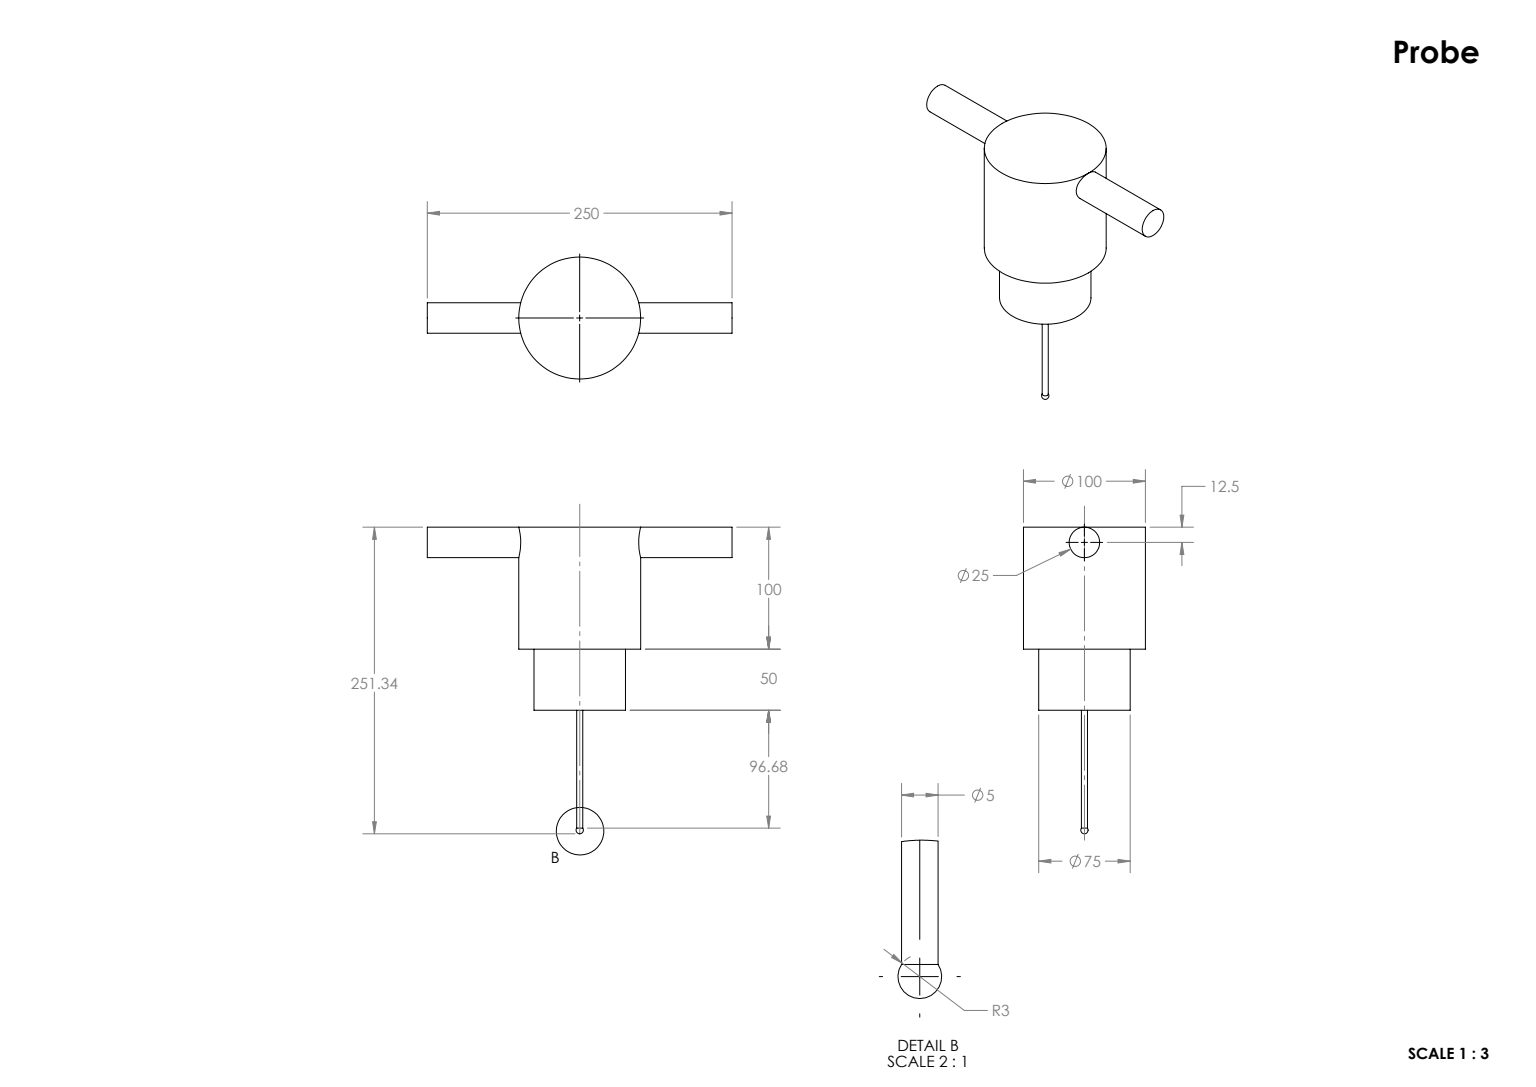
ISO-10303-21;
HEADER;
FILE_DESCRIPTION (('STEP AP214'),
    '1' );
FILE_NAME ('Probe.step',
    '2026-10-28T15:55:38',
    ( '' ),
    ( '' ),
    'SwSTEP 2.0',
    'SolidWorks 2025',
    '' );
FILE_SCHEMA (( 'AUTOMOTIVE_DESIGN' ));
ENDSEC;

DATA;
#19=ADVANCED_FACE ( 'NONE', ( #8129 ), #7501, .T. ) ;
#39=CARTESIAN_POINT ( 'NONE',  ( 0.000000000000000000, 7.945337353457666419E-16, -150.0000000000000000 ) ) ;
#48=VERTEX_POINT ( 'NONE', #4805 ) ;
#114=CARTESIAN_POINT ( 'NONE',  ( -0.8292248493948853882, 50.00000000000000000, -1.010867942207665278E-14 ) ) ;
#115=FACE_OUTER_BOUND ( 'NONE', #7634, .T. ) ;
#118=DIRECTION ( 'NONE',  ( 0.000000000000000000, 0.000000000000000000, -1.000000000000000000 ) ) ;
#135=EDGE_CURVE ( 'NONE', #3598, #1656, #3145, .T. ) ;
#154=CARTESIAN_POINT ( 'NONE',  ( -5.558076868459232323, 49.69586384218322905, -1.274058936613796877 ) ) ;
#176=LINE ( 'NONE', #2239, #1981 ) ;
#182=ORIENTED_EDGE ( 'NONE', *, *, #917, .F. ) ;
#188=ADVANCED_FACE ( 'NONE', ( #4425 ), #4987, .T. ) ;
#201=DIRECTION ( 'NONE',  ( 0.000000000000000000, -0.000000000000000000, 1.000000000000000000 ) ) ;
#222=AXIS2_PLACEMENT_3D ( 'NONE', #4618, #3222, #5811 ) ;
#242=CARTESIAN_POINT ( 'NONE',  ( 8.253058034503027329, 49.31520865873546455, -3.102932425833026642 ) ) ;
#263=DIRECTION ( 'NONE',  ( -0.000000000000000000, -7.945337353457666666E-18, -1.000000000000000000 ) ) ;
#281=CARTESIAN_POINT ( 'NONE',  ( 0.000000000000000000, 50.00000000000000000, 0.000000000000000000 ) ) ;
#307=PLANE ( 'NONE',  #7987 ) ;
#327=CARTESIAN_POINT ( 'NONE',  ( 11.38744771879169093, 48.68625849413228934, -7.328777110660809946 ) ) ;
#334=VERTEX_POINT ( 'NONE', #4039 ) ;
#341=CARTESIAN_POINT ( 'NONE',  ( -8.253058034503022000, -49.31520865873545034, -3.102932425833025309 ) ) ;
#392=ORIENTED_EDGE ( 'NONE', *, *, #1590, .F. ) ;
#401=CARTESIAN_POINT ( 'NONE',  ( 1.632468168883557169, -49.97996006834705440, -24.92059050027006606 ) ) ;
#418=ORIENTED_EDGE ( 'NONE', *, *, #1413, .T. ) ;
#423=CARTESIAN_POINT ( 'NONE',  ( 0.000000000000000000, 1.191800603018649864E-15, -100.0000000000000000 ) ) ;
#435=EDGE_LOOP ( 'NONE', ( #3516, #6927 ) ) ;
#446=ORIENTED_EDGE ( 'NONE', *, *, #1545, .T. ) ;
#457=AXIS2_PLACEMENT_3D ( 'NONE', #8109, #6795, #201 ) ;
#479=CARTESIAN_POINT ( 'NONE',  ( -11.83759003446072811, -48.57866412327431505, -8.463974912767858072 ) ) ;
#484=CARTESIAN_POINT ( 'NONE',  ( 0.000000000000000000, 37.49999999999999289, -150.0000000000000000 ) ) ;
#491=UNCERTAINTY_MEASURE_WITH_UNIT (LENGTH_MEASURE( 1.000000000000000082E-05 ), #6982, 'distance_accuracy_value', 'NONE');
#496=ADVANCED_FACE ( 'NONE', ( #6675 ), #5448, .T. ) ;
#505=EDGE_CURVE ( 'NONE', #48, #4486, #8022, .T. ) ;
#522=CARTESIAN_POINT ( 'NONE',  ( -3.257728639534228865, -49.90026920665918198, -24.59591892738197672 ) ) ;
#526=CARTESIAN_POINT ( 'NONE',  ( 0.000000000000000000, 7.945337353457666419E-16, -150.0000000000000000 ) ) ;
#533=CARTESIAN_POINT ( 'NONE',  ( 11.22541203495697104, -48.72469304432832615, -18.06039341770851436 ) ) ;
#551=CARTESIAN_POINT ( 'NONE',  ( 12.41819479434714069, 48.43362276422629975, -14.14586790793774895 ) ) ;
#558=CARTESIAN_POINT ( 'NONE',  ( -9.403142016537936243, 49.10855715295182478, -4.253968596005561764 ) ) ;
#573=SHAPE_REPRESENTATION ( 'Probe', ( #1299 ), #7094 ) ;
#575=CARTESIAN_POINT ( 'NONE',  ( 9.403142016537936243, -49.10855715295183188, -4.253968596005562652 ) ) ;
#592=CARTESIAN_POINT ( 'NONE',  ( 4.037232620646171277, 49.84250566375262537, -24.35825330067164884 ) ) ;
#595=DIRECTION ( 'NONE',  ( 0.000000000000000000, 1.000000000000000000, 0.000000000000000000 ) ) ;
#618=CARTESIAN_POINT ( 'NONE',  ( 12.39753912377990552, -48.43864980223353456, -14.14916085730400219 ) ) ;
#640=DIRECTION ( 'NONE',  ( 0.000000000000000000, -7.945337353457666666E-18, -1.000000000000000000 ) ) ;
#658=CARTESIAN_POINT ( 'NONE',  ( 10.16267929626374489, -48.95685099404312979, -19.78936650929338725 ) ) ;
#661=FACE_OUTER_BOUND ( 'NONE', #6204, .T. ) ;
#662=ORIENTED_EDGE ( 'NONE', *, *, #737, .F. ) ;
#680=EDGE_CURVE ( 'NONE', #1656, #1706, #2751, .T. ) ;
#702=CARTESIAN_POINT ( 'NONE',  ( 6.614448519079572542, -49.56174273647120998, -23.11440585317444985 ) ) ;
#721=EDGE_CURVE ( 'NONE', #7126, #7967, #3963, .T. ) ;
#737=EDGE_CURVE ( 'NONE', #986, #5147, #4224, .T. ) ;
#739=ORIENTED_EDGE ( 'NONE', *, *, #1590, .T. ) ;
#742=VECTOR ( 'NONE', #864, 1000.000000000000000 ) ;
#775=ORIENTED_EDGE ( 'NONE', *, *, #5713, .F. ) ;
#781=DIRECTION ( 'NONE',  ( -0.000000000000000000, -7.945337353457666666E-18, -1.000000000000000000 ) ) ;
#791=DIRECTION ( 'NONE',  ( 0.000000000000000000, 1.000000000000000000, -7.945337353457666666E-18 ) ) ;
#843=EDGE_LOOP ( 'NONE', ( #1832, #4978 ) ) ;
#856=ORIENTED_EDGE ( 'NONE', *, *, #2130, .F. ) ;
#861=DIRECTION ( 'NONE',  ( 0.000000000000000000, 0.000000000000000000, -1.000000000000000000 ) ) ;
#864=DIRECTION ( 'NONE',  ( -0.000000000000000000, -7.945337353457666666E-18, -1.000000000000000000 ) ) ;
#908=CARTESIAN_POINT ( 'NONE',  ( 6.123233995736765296E-15, -49.99999999999999289, -250.0000000000000000 ) ) ;
#917=EDGE_CURVE ( 'NONE', #6329, #7967, #176, .T. ) ;
#918=AXIS2_PLACEMENT_3D ( 'NONE', #7982, #6026, #118 ) ;
#936=CARTESIAN_POINT ( 'NONE',  ( 9.415432556623352767, 49.10895683582204896, -4.238112224658974192 ) ) ;
#941=DIRECTION ( 'NONE',  ( -0.000000000000000000, -7.945337353457666666E-18, -1.000000000000000000 ) ) ;
#986=VERTEX_POINT ( 'NONE', #3576 ) ;
#987=AXIS2_PLACEMENT_3D ( 'NONE', #3005, #4347, #3590 ) ;
#993=CARTESIAN_POINT ( 'NONE',  ( -3.243174531372579494, -49.89626761698126245, -0.4210505255250470702 ) ) ;
#996=ORIENTED_EDGE ( 'NONE', *, *, #4675, .T. ) ;
#997=DIRECTION ( 'NONE',  ( -0.000000000000000000, -7.945337353457666666E-18, -1.000000000000000000 ) ) ;
#1024=EDGE_CURVE ( 'NONE', #3915, #6928, #8311, .T. ) ;
#1028=AXIS2_PLACEMENT_3D ( 'NONE', #3244, #2009, #3886 ) ;
#1035=DIRECTION ( 'NONE',  ( 0.000000000000000000, 1.000000000000000000, 0.000000000000000000 ) ) ;
#1043=CARTESIAN_POINT ( 'NONE',  ( 6.123246359811209136E-15, -49.99999999999999289, -25.00000000000000000 ) ) ;
#1058=CARTESIAN_POINT ( 'NONE',  ( 10.82846484896509409, 48.81376096915064267, -6.242155733168283760 ) ) ;
#1069=ORIENTED_EDGE ( 'NONE', *, *, #2887, .T. ) ;
#1072=CIRCLE ( 'NONE', #2296, 49.99999999999998579 ) ;
#1077=CARTESIAN_POINT ( 'NONE',  ( -6.271675211807169248, -49.60982880777383741, -1.656483108071704846 ) ) ;
#1130=DIRECTION ( 'NONE',  ( -0.000000000000000000, -7.945337353457666666E-18, -1.000000000000000000 ) ) ;
#1150=ORIENTED_EDGE ( 'NONE', *, *, #1915, .F. ) ;
#1154=CARTESIAN_POINT ( 'NONE',  ( -12.41973075191816633, 48.43322590808264039, -10.86594944112156291 ) ) ;
#1157=ADVANCED_FACE ( 'NONE', ( #2546 ), #4549, .F. ) ;
#1171=CARTESIAN_POINT ( 'NONE',  ( 8.557270319823464533, -49.26314968593496957, -3.379276828450694214 ) ) ;
#1190=CIRCLE ( 'NONE', #5890, 37.49999999999999289 ) ;
#1198=CARTESIAN_POINT ( 'NONE',  ( -12.10063575899649813, 48.51393303002350166, -9.260486547765557575 ) ) ;
#1203=FACE_OUTER_BOUND ( 'NONE', #1797, .T. ) ;
#1234=EDGE_LOOP ( 'NONE', ( #2994, #6172, #2615, #1150, #7419, #6336 ) ) ;
#1237=ADVANCED_FACE ( 'NONE', ( #115 ), #2704, .T. ) ;
#1240=CARTESIAN_POINT ( 'NONE',  ( -8.256742446866505603, 49.31458024324043521, -3.106261761854182790 ) ) ;
#1254=AXIS2_PLACEMENT_3D ( 'NONE', #7140, #640, #1365 ) ;
#1256=DIRECTION ( 'NONE',  ( -0.000000000000000000, -7.945337353457666666E-18, -1.000000000000000000 ) ) ;
#1274=CARTESIAN_POINT ( 'NONE',  ( -11.69966253144281332, 48.61218256317027198, -16.92010850872651417 ) ) ;
#1299=AXIS2_PLACEMENT_3D ( 'NONE', #5884, #1507, #5927 ) ;
#1319=DIRECTION ( 'NONE',  ( 0.000000000000000000, 1.000000000000000000, -7.945337353457666666E-18 ) ) ;
#1320=DIRECTION ( 'NONE',  ( -0.000000000000000000, -7.945337353457666666E-18, -1.000000000000000000 ) ) ;
#1330=CIRCLE ( 'NONE', #1730, 37.50000000000000000 ) ;
#1333=AXIS2_PLACEMENT_3D ( 'NONE', #3199, #3801, #595 ) ;
#1336=CARTESIAN_POINT ( 'NONE',  ( 3.061616997868370815E-16, -2.499999999999990230, -250.0000000000000000 ) ) ;
#1365=DIRECTION ( 'NONE',  ( 0.000000000000000000, 1.000000000000000000, -7.945337353457666666E-18 ) ) ;
#1384=DIRECTION ( 'NONE',  ( 0.000000000000000000, 1.000000000000000000, 0.000000000000000000 ) ) ;
#1412=VECTOR ( 'NONE', #1613, 1000.000000000000000 ) ;
#1413=EDGE_CURVE ( 'NONE', #5147, #4486, #4874, .T. ) ;
#1437=ADVANCED_FACE ( 'NONE', ( #7243, #6733 ), #307, .T. ) ;
#1502=FACE_OUTER_BOUND ( 'NONE', #1234, .T. ) ;
#1507=DIRECTION ( 'NONE',  ( 0.000000000000000000, 0.000000000000000000, 1.000000000000000000 ) ) ;
#1524=CARTESIAN_POINT ( 'NONE',  ( -6.274835263354055392, 49.60946935866542162, -1.658027691731842168 ) ) ;
#1527=DIRECTION ( 'NONE',  ( 0.000000000000000000, 1.000000000000000000, 0.000000000000000000 ) ) ;
#1540=DIRECTION ( 'NONE',  ( 0.000000000000000000, 1.000000000000000000, 0.000000000000000000 ) ) ;
#1545=EDGE_CURVE ( 'NONE', #6928, #3915, #4197, .T. ) ;
#1582=CARTESIAN_POINT ( 'NONE',  ( -11.21042436406065868, -48.72746226073034137, -18.04468079945885250 ) ) ;
#1590=EDGE_CURVE ( 'NONE', #4209, #6887, #3943, .T. ) ;
#1613=DIRECTION ( 'NONE',  ( -0.000000000000000000, -1.000000000000000000, -0.000000000000000000 ) ) ;
#1627=CARTESIAN_POINT ( 'NONE',  ( -0.8294483708339484007, -50.00000000000000711, -7.623296525288703052E-18 ) ) ;
#1641=ORIENTED_EDGE ( 'NONE', *, *, #4698, .F. ) ;
#1653=CARTESIAN_POINT ( 'NONE',  ( 0.000000000000000000, -125.0000000000000000, -12.50000000000000000 ) ) ;
#1655=EDGE_CURVE ( 'NONE', #6306, #986, #7595, .T. ) ;
#1656=VERTEX_POINT ( 'NONE', #5197 ) ;
#1706=VERTEX_POINT ( 'NONE', #4397 ) ;
#1707=CARTESIAN_POINT ( 'NONE',  ( -12.09737906851130518, -48.51474822866212122, -15.75174765218248574 ) ) ;
#1730=AXIS2_PLACEMENT_3D ( 'NONE', #423, #3269, #2425 ) ;
#1746=EDGE_LOOP ( 'NONE', ( #2201, #2378 ) ) ;
#1747=EDGE_LOOP ( 'NONE', ( #5047, #7771, #6216, #6700 ) ) ;
#1770=CARTESIAN_POINT ( 'NONE',  ( 6.260380647299085055, -49.60786550102538683, -23.32709356835264103 ) ) ;
#1772=CARTESIAN_POINT ( 'NONE',  ( 0.000000000000000000, 0.000000000000000000, -248.3416876048222832 ) ) ;
#1781=CARTESIAN_POINT ( 'NONE',  ( 9.126495132297687718, 49.16089547422080130, -21.05129937300930010 ) ) ;
#1797=EDGE_LOOP ( 'NONE', ( #6153, #2426, #2650, #2275 ) ) ;
#1798=CARTESIAN_POINT ( 'NONE',  ( -0.4088724290315628451, -49.99999999999999289, -25.00000000000000000 ) ) ;
#1813=SPHERICAL_SURFACE ( 'NONE', #3588, 3.000000000000001776 ) ;
#1832=ORIENTED_EDGE ( 'NONE', *, *, #6250, .F. ) ;
#1835=CARTESIAN_POINT ( 'NONE',  ( -9.920070434648176061, 49.00675803034337008, -20.11641848348689976 ) ) ;
#1838=DIRECTION ( 'NONE',  ( 0.000000000000000000, 0.000000000000000000, -1.000000000000000000 ) ) ;
#1846=CARTESIAN_POINT ( 'NONE',  ( 12.10063575899649990, -48.51393303002349455, -9.260486547765564680 ) ) ;
#1865=CARTESIAN_POINT ( 'NONE',  ( 7.630101673356683101, 49.41909675622682840, -22.43442449636368252 ) ) ;
#1879=CARTESIAN_POINT ( 'NONE',  ( -6.260380647299085055, 49.60786550102537973, -23.32709356835263748 ) ) ;
#1881=CIRCLE ( 'NONE', #1333, 2.499999999999984013 ) ;
#1885=DIRECTION ( 'NONE',  ( -0.000000000000000000, -1.000000000000000000, -0.000000000000000000 ) ) ;
#1888=CARTESIAN_POINT ( 'NONE',  ( 0.000000000000000000, -1.262567713204993255E-33, -150.0000000000000000 ) ) ;
#1890=CARTESIAN_POINT ( 'NONE',  ( -10.16275934324372265, -48.95683464664497819, -19.78926114801198821 ) ) ;
#1895=CYLINDRICAL_SURFACE ( 'NONE', #4148, 37.49999999999999289 ) ;
#1896=CARTESIAN_POINT ( 'NONE',  ( 12.07731880710695904, -48.51961889015784379, -15.74894529186713577 ) ) ;
#1912=CARTESIAN_POINT ( 'NONE',  ( 0.4088724290315675081, 49.99999999999999289, -24.99999999999999645 ) ) ;
#1915=EDGE_CURVE ( 'NONE', #6329, #6306, #3408, .T. ) ;
#1923=CARTESIAN_POINT ( 'NONE',  ( -9.123515037571456432, 49.16144051280856786, -21.05438506594878945 ) ) ;
#1947=CARTESIAN_POINT ( 'NONE',  ( 0.000000000000000000, -125.0000000000000000, -12.50000000000000000 ) ) ;
#1957=CARTESIAN_POINT ( 'NONE',  ( 12.50034226774477730, 48.41220345444930473, -13.31371842734950839 ) ) ;
#1971=LINE ( 'NONE', #3126, #6847 ) ;
#1975=CARTESIAN_POINT ( 'NONE',  ( -8.257771144136533792, -49.31688802671483529, -21.91964719072836232 ) ) ;
#1981=VECTOR ( 'NONE', #4658, 1000.000000000000000 ) ;
#2009=DIRECTION ( 'NONE',  ( 0.000000000000000000, 1.000000000000000000, 0.000000000000000000 ) ) ;
#2027=AXIS2_PLACEMENT_3D ( 'NONE', #3385, #5895, #2157 ) ;
#2037=AXIS2_PLACEMENT_3D ( 'NONE', #3347, #2118, #2154 ) ;
#2043=VECTOR ( 'NONE', #2971, 1000.000000000000000 ) ;
#2071=EDGE_LOOP ( 'NONE', ( #4525, #6589, #7855 ) ) ;
#2090=AXIS2_PLACEMENT_3D ( 'NONE', #4600, #2777, #1319 ) ;
#2118=DIRECTION ( 'NONE',  ( -0.000000000000000000, -7.945337353457666666E-18, -1.000000000000000000 ) ) ;
#2130=EDGE_CURVE ( 'NONE', #6306, #6329, #5453, .T. ) ;
#2143=CARTESIAN_POINT ( 'NONE',  ( 0.000000000000000000, 0.000000000000000000, -250.0000000000000000 ) ) ;
#2154=DIRECTION ( 'NONE',  ( 0.000000000000000000, 1.000000000000000000, -7.945337353457666666E-18 ) ) ;
#2157=DIRECTION ( 'NONE',  ( 0.000000000000000000, 0.000000000000000000, -1.000000000000000000 ) ) ;
#2185=DIRECTION ( 'NONE',  ( -0.000000000000000000, -1.000000000000000000, -0.000000000000000000 ) ) ;
#2201=ORIENTED_EDGE ( 'NONE', *, *, #135, .F. ) ;
#2213=DIRECTION ( 'NONE',  ( -0.000000000000000000, -7.945337353457666666E-18, -1.000000000000000000 ) ) ;
#2236=CARTESIAN_POINT ( 'NONE',  ( -12.41819479434713891, -48.43362276422628554, -14.14586790793774895 ) ) ;
#2237=SHAPE_REPRESENTATION_RELATIONSHIP ( 'NONE' , 'NONE' ,  #573, #6521 ) ;
#2239=CARTESIAN_POINT ( 'NONE',  ( 0.000000000000000000, 49.99999999999999289, -250.0000000000000000 ) ) ;
#2250=CARTESIAN_POINT ( 'NONE',  ( 0.000000000000000000, 1.191800603018649864E-15, -100.0000000000000000 ) ) ;
#2256=DIRECTION ( 'NONE',  ( 1.000000000000000000, -0.000000000000000000, 0.000000000000000000 ) ) ;
#2275=ORIENTED_EDGE ( 'NONE', *, *, #7081, .F. ) ;
#2296=AXIS2_PLACEMENT_3D ( 'NONE', #6352, #1256, #5080 ) ;
#2310=CARTESIAN_POINT ( 'NONE',  ( -12.07658505203027843, -48.51980254810341364, -9.248211290718611366 ) ) ;
#2350=CARTESIAN_POINT ( 'NONE',  ( -2.846087801003401196, -49.92054308009031161, -0.3214687869884009230 ) ) ;
#2351=( LENGTH_UNIT ( ) NAMED_UNIT ( * ) SI_UNIT ( .MILLI., .METRE. ) );
#2378=ORIENTED_EDGE ( 'NONE', *, *, #2977, .F. ) ;
#2391=CARTESIAN_POINT ( 'NONE',  ( -8.554558110533214688, -49.26362287191481215, -3.376715202643650215 ) ) ;
#2414=AXIS2_PLACEMENT_3D ( 'NONE', #3771, #1320, #7059 ) ;
#2418=CARTESIAN_POINT ( 'NONE',  ( 5.169052467613985513, 49.73353547763981908, -23.88849205255369412 ) ) ;
#2425=DIRECTION ( 'NONE',  ( 0.000000000000000000, 1.000000000000000000, 0.000000000000000000 ) ) ;
#2426=ORIENTED_EDGE ( 'NONE', *, *, #680, .T. ) ;
#2462=CARTESIAN_POINT ( 'NONE',  ( 12.07658505203027843, 48.51980254810342075, -9.248211290718606037 ) ) ;
#2470=DIRECTION ( 'NONE',  ( -0.000000000000000000, -7.945337353457666666E-18, -1.000000000000000000 ) ) ;
#2486=CARTESIAN_POINT ( 'NONE',  ( 9.123515037571451103, -49.16144051280858207, -21.05438506594878234 ) ) ;
#2501=CARTESIAN_POINT ( 'NONE',  ( 12.41960978562214102, 48.43326235599739960, -10.86247626165360813 ) ) ;
#2506=CARTESIAN_POINT ( 'NONE',  ( -11.83910760917652460, 48.57829327830486221, -16.53147691254502760 ) ) ;
#2507=ORIENTED_EDGE ( 'NONE', *, *, #5064, .T. ) ;
#2546=FACE_OUTER_BOUND ( 'NONE', #6856, .T. ) ;
#2563=CARTESIAN_POINT ( 'NONE',  ( 9.920070434648168956, -49.00675803034337719, -20.11641848348691042 ) ) ;
#2564=VECTOR ( 'NONE', #6472, 1000.000000000000000 ) ;
#2578=ADVANCED_FACE ( 'NONE', ( #4354 ), #1813, .T. ) ;
#2581=CARTESIAN_POINT ( 'NONE',  ( 10.16275934324372621, 48.95683464664498530, -19.78926114801199532 ) ) ;
#2598=CARTESIAN_POINT ( 'NONE',  ( -0.8183949479883554368, -49.99498560413270809, -24.97998898815200874 ) ) ;
#2615=ORIENTED_EDGE ( 'NONE', *, *, #5679, .T. ) ;
#2643=CARTESIAN_POINT ( 'NONE',  ( 8.258796090566862702, -49.31668406204209276, -21.91840799305901299 ) ) ;
#2647=ORIENTED_EDGE ( 'NONE', *, *, #8043, .T. ) ;
#2650=ORIENTED_EDGE ( 'NONE', *, *, #8282, .F. ) ;
#2690=DIRECTION ( 'NONE',  ( -1.000000000000000000, -1.224646799147353207E-16, 9.730231958057834423E-34 ) ) ;
#2692=CIRCLE ( 'NONE', #3349, 12.50000000000000000 ) ;
#2694=FACE_OUTER_BOUND ( 'NONE', #3875, .T. ) ;
#2698=VECTOR ( 'NONE', #7949, 1000.000000000000000 ) ;
#2704=CYLINDRICAL_SURFACE ( 'NONE', #6225, 2.499999999999990230 ) ;
#2710=ORIENTED_EDGE ( 'NONE', *, *, #6560, .T. ) ;
#2715=ADVANCED_FACE ( 'NONE', ( #661 ), #7879, .T. ) ;
#2751=LINE ( 'NONE', #7916, #742 ) ;
#2761=EDGE_LOOP ( 'NONE', ( #662, #5308, #3301, #6052 ) ) ;
#2777=DIRECTION ( 'NONE',  ( -0.000000000000000000, -7.945337353457666666E-18, -1.000000000000000000 ) ) ;
#2786=ORIENTED_EDGE ( 'NONE', *, *, #4582, .F. ) ;
#2803=VERTEX_POINT ( 'NONE', #7962 ) ;
#2820=CARTESIAN_POINT ( 'NONE',  ( 8.554558110533218240, 49.26362287191481926, -3.376715202643651992 ) ) ;
#2830=B_SPLINE_CURVE_WITH_KNOTS ( 'NONE', 3,
 ( #1043, #3597, #401, #7500, #4263, #6264, #3644, #1770, #702, #5767, #2643, #2486, #5683, #2563, #658, #4481, #533, #7033, #6353, #1896, #4352, #6426, #618, #5126, #7071, #3258, #3218, #1846, #5848, #5081, #7116, #3177, #5212, #575, #3784, #1171, #5809, #7726, #3736, #7631, #3106, #7764, #6313, #5043, #8266, #4440, #4391, #3860 ),
 .UNSPECIFIED., .F., .F.,
 ( 4, 2, 2, 2, 2, 2, 2, 2, 2, 2, 2, 2, 2, 2, 2, 2, 2, 2, 2, 2, 2, 2, 2, 4 ),
 ( 0.03923685324657889828, 0.04168849572278653104, 0.04414013819899415686, 0.04536595943709797324, 0.04659178067520178962, 0.04904342315140942932, 0.05026924438951324570, 0.05149506562761706902, 0.05394670810382472259, 0.05517252934192855285, 0.05639835058003237617, 0.05762417181813619949, 0.05884999305624002280, 0.06130163553244767638, 0.06375327800865532302, 0.06620492048486296965, 0.06743074172296678603, 0.06865656296107061629, 0.06988238419917444655, 0.07110820543727826293, 0.07355984791348590957, 0.07478566915158973982, 0.07601149038969357008, 0.07846313286590121672 ),
 .UNSPECIFIED. ) ;
#2875=LINE ( 'NONE', #908, #4393 ) ;
#2887=EDGE_CURVE ( 'NONE', #48, #7126, #2875, .T. ) ;
#2896=CARTESIAN_POINT ( 'NONE',  ( 4.420576121828488247, 49.80565028682020312, -0.8005904993895475164 ) ) ;
#2901=STYLED_ITEM('',(#8393),#3583);
#2916=AXIS2_PLACEMENT_3D ( 'NONE', #2143, #781, #3334 ) ;
#2933=PRODUCT_DEFINITION_CONTEXT ( 'detailed design', #5219, 'design' ) ;
#2944=CARTESIAN_POINT ( 'NONE',  ( 0.8294483708339475125, 49.99999999999998579, -1.039817646049378781E-14 ) ) ;
#2960=( NAMED_UNIT ( * ) SI_UNIT ( $, .STERADIAN. ) SOLID_ANGLE_UNIT ( ) );
#2971=DIRECTION ( 'NONE',  ( -0.000000000000000000, -7.945337353457666666E-18, -1.000000000000000000 ) ) ;
#2977=EDGE_CURVE ( 'NONE', #1656, #3598, #1330, .T. ) ;
#2994=ORIENTED_EDGE ( 'NONE', *, *, #2887, .F. ) ;
#2999=FACE_OUTER_BOUND ( 'NONE', #5824, .T. ) ;
#3001=CARTESIAN_POINT ( 'NONE',  ( 0.000000000000000000, -49.99999999999999289, 0.000000000000000000 ) ) ;
#3005=CARTESIAN_POINT ( 'NONE',  ( 0.000000000000000000, 125.0000000000000000, -12.50000000000000000 ) ) ;
#3020=DIRECTION ( 'NONE',  ( 0.000000000000000000, 0.000000000000000000, -1.000000000000000000 ) ) ;
#3025=ADVANCED_FACE ( 'NONE', ( #7522 ), #4933, .F. ) ;
#3046=CARTESIAN_POINT ( 'NONE',  ( -7.630101673356672443, -49.41909675622684261, -22.43442449636368607 ) ) ;
#3073=CARTESIAN_POINT ( 'NONE',  ( 3.257728639534230197, 49.90026920665918198, -24.59591892738197672 ) ) ;
#3087=CARTESIAN_POINT ( 'NONE',  ( -10.16604137791875750, 48.95616179457642403, -5.215114234092023793 ) ) ;
#3095=CARTESIAN_POINT ( 'NONE',  ( -10.82421258667007891, -48.81470695058813902, -18.76526308057255932 ) ) ;
#3106=CARTESIAN_POINT ( 'NONE',  ( 5.558076868459242981, -49.69586384218322905, -1.274058936613802651 ) ) ;
#3110=UNCERTAINTY_MEASURE_WITH_UNIT (LENGTH_MEASURE( 1.000000000000000082E-05 ), #2351, 'distance_accuracy_value', 'NONE');
#3118=CARTESIAN_POINT ( 'NONE',  ( 11.86014387961076011, 48.57408496170469192, -16.53260109561406566 ) ) ;
#3123=CARTESIAN_POINT ( 'NONE',  ( -10.84023063519268604, 48.81293515762427404, -18.77686690299335126 ) ) ;
#3126=CARTESIAN_POINT ( 'NONE',  ( 1.530808498934191521E-15, 125.0000000000000000, 0.000000000000000000 ) ) ;
#3131=CARTESIAN_POINT ( 'NONE',  ( -10.61457161467472865, -48.86086578770956379, -19.11406644883055961 ) ) ;
#3142=CARTESIAN_POINT ( 'NONE',  ( 11.83759003446072455, 48.57866412327430794, -8.463974912767849190 ) ) ;
#3145=CIRCLE ( 'NONE', #3531, 37.50000000000000000 ) ;
#3147=ORIENTED_EDGE ( 'NONE', *, *, #3367, .F. ) ;
#3164=CARTESIAN_POINT ( 'NONE',  ( -1.236408833568031405E-20, 49.99999999999999289, -25.00000000000000000 ) ) ;
#3165=DIRECTION ( 'NONE',  ( -0.000000000000000000, -7.945337353457666666E-18, -1.000000000000000000 ) ) ;
#3177=CARTESIAN_POINT ( 'NONE',  ( 10.16604137791875573, -48.95616179457642403, -5.215114234092022905 ) ) ;
#3194=CARTESIAN_POINT ( 'NONE',  ( 11.21042436406066578, 48.72746226073035558, -18.04468079945885250 ) ) ;
#3199=CARTESIAN_POINT ( 'NONE',  ( 0.000000000000000000, 2.635170283421476540E-17, -246.6833752096445664 ) ) ;
#3205=CARTESIAN_POINT ( 'NONE',  ( -8.258796090566862702, 49.31668406204208566, -21.91840799305900589 ) ) ;
#3218=CARTESIAN_POINT ( 'NONE',  ( 12.41973075191816811, -48.43322590808266170, -10.86594944112157535 ) ) ;
#3222=DIRECTION ( 'NONE',  ( -1.000000000000000000, -0.000000000000000000, 0.000000000000000000 ) ) ;
#3243=CARTESIAN_POINT ( 'NONE',  ( -12.17681684015966681, 48.49465898589869539, -15.35333092327343429 ) ) ;
#3244=CARTESIAN_POINT ( 'NONE',  ( 0.000000000000000000, 125.0000000000000000, -12.50000000000000000 ) ) ;
#3258=CARTESIAN_POINT ( 'NONE',  ( 12.50025679328619788, -48.41222552385477940, -11.67941733774923030 ) ) ;
#3269=DIRECTION ( 'NONE',  ( -0.000000000000000000, -7.945337353457666666E-18, -1.000000000000000000 ) ) ;
#3281=CARTESIAN_POINT ( 'NONE',  ( -7.296436711415922538, 49.46595054402523317, -2.342244756090384961 ) ) ;
#3301=ORIENTED_EDGE ( 'NONE', *, *, #505, .T. ) ;
#3312=ORIENTED_EDGE ( 'NONE', *, *, #505, .F. ) ;
#3317=CARTESIAN_POINT ( 'NONE',  ( -4.044723210857149809, 49.83770199522208344, -0.6652966195906341307 ) ) ;
#3334=DIRECTION ( 'NONE',  ( 0.000000000000000000, 1.000000000000000000, 0.000000000000000000 ) ) ;
#3347=CARTESIAN_POINT ( 'NONE',  ( 0.000000000000000000, 1.986334338364416506E-15, 0.000000000000000000 ) ) ;
#3349=AXIS2_PLACEMENT_3D ( 'NONE', #1653, #7485, #6205 ) ;
#3367=EDGE_CURVE ( 'NONE', #48, #986, #2830, .T. ) ;
#3381=ORIENTED_EDGE ( 'NONE', *, *, #7081, .T. ) ;
#3383=CARTESIAN_POINT ( 'NONE',  ( 0.000000000000000000, 0.000000000000000000, -248.3416876048222832 ) ) ;
#3385=CARTESIAN_POINT ( 'NONE',  ( 0.000000000000000000, 125.0000000000000000, -12.50000000000000000 ) ) ;
#3398=CARTESIAN_POINT ( 'NONE',  ( 0.000000000000000000, 125.0000000000000000, -25.00000000000000000 ) ) ;
#3408=B_SPLINE_CURVE_WITH_KNOTS ( 'NONE', 3,
 ( #3164, #4502, #5110, #3842, #7095, #4423, #4378, #1879, #7707, #4466, #3205, #1923, #7053, #1835, #6407, #3123, #8248, #1274, #2506, #5154, #3243, #7614, #6457, #5705, #8201, #7017, #1154, #1198, #3767, #3716, #6290, #3087, #5669, #558, #5066, #7659, #1240, #4546, #3281, #1524, #154, #7905, #3317, #5868, #5905, #4641, #114, #7939 ),
 .UNSPECIFIED., .F., .F.,
 ( 4, 2, 2, 2, 2, 2, 2, 2, 2, 2, 2, 2, 2, 2, 2, 2, 2, 2, 2, 2, 2, 2, 2, 4 ),
 ( 0.03923685324657887746, 0.04168849572278652410, 0.04414013819899417074, 0.04536595943709799406, 0.04659178067520181737, 0.04904342315140946401, 0.05026924438951328733, 0.05149506562761710371, 0.05394670810382474341, 0.05517252934192855979, 0.05639835058003238311, 0.05762417181813619949, 0.05884999305624001587, 0.06130163553244766250, 0.06375327800865530914, 0.06620492048486295578, 0.06743074172296677216, 0.06865656296107058854, 0.06988238419917441879, 0.07110820543727824905, 0.07355984791348588181, 0.07478566915158971207, 0.07601149038969352845, 0.07846313286590117508 ),
 .UNSPECIFIED. ) ;
#3410=PRODUCT_DEFINITION_SHAPE ( 'NONE', 'NONE',  #4147 ) ;
#3441=CYLINDRICAL_SURFACE ( 'NONE', #918, 12.50000000000000000 ) ;
#3443=CARTESIAN_POINT ( 'NONE',  ( 0.000000000000000000, 125.0000000000000000, -25.00000000000000000 ) ) ;
#3469=DIRECTION ( 'NONE',  ( -0.000000000000000000, -7.945337353457666666E-18, -1.000000000000000000 ) ) ;
#3510=DIRECTION ( 'NONE',  ( -0.000000000000000000, -1.000000000000000000, -0.000000000000000000 ) ) ;
#3516=ORIENTED_EDGE ( 'NONE', *, *, #7217, .T. ) ;
#3520=CARTESIAN_POINT ( 'NONE',  ( 10.61691938675656566, 48.86036797030515544, -5.889423163904315750 ) ) ;
#3524=PRODUCT_DEFINITION_FORMATION_WITH_SPECIFIED_SOURCE ( 'ANY', '', #5324, .NOT_KNOWN. ) ;
#3531=AXIS2_PLACEMENT_3D ( 'NONE', #4684, #7397, #4725 ) ;
#3539=CARTESIAN_POINT ( 'NONE',  ( -10.61691938675656921, -48.86036797030517675, -5.889423163904312197 ) ) ;
#3547=EDGE_CURVE ( 'NONE', #986, #48, #4231, .T. ) ;
#3576=CARTESIAN_POINT ( 'NONE',  ( 0.000000000000000000, -49.99999999999999289, 0.000000000000000000 ) ) ;
#3582=CARTESIAN_POINT ( 'NONE',  ( -9.415432556623350990, -49.10895683582203475, -4.238112224658973304 ) ) ;
#3583=MANIFOLD_SOLID_BREP ( 'Boss-Extrude1', #6653 ) ;
#3588=AXIS2_PLACEMENT_3D ( 'NONE', #1772, #5601, #6318 ) ;
#3590=DIRECTION ( 'NONE',  ( 0.000000000000000000, 0.000000000000000000, 1.000000000000000000 ) ) ;
#3597=CARTESIAN_POINT ( 'NONE',  ( 0.8175244905105739646, -49.99999999999999289, -25.00000000000000355 ) ) ;
#3598=VERTEX_POINT ( 'NONE', #5119 ) ;
#3611=CARTESIAN_POINT ( 'NONE',  ( 1.644392415218296488, 49.97938897499116706, -0.08173415109641088416 ) ) ;
#3631=CARTESIAN_POINT ( 'NONE',  ( -11.38744771879169093, -48.68625849413228934, -7.328777110660809058 ) ) ;
#3644=CARTESIAN_POINT ( 'NONE',  ( 5.536947881659092019, -49.69381142126947992, -23.71430020744633893 ) ) ;
#3679=CARTESIAN_POINT ( 'NONE',  ( -7.620025376658135841, -49.41698073774416144, -2.582688914155140125 ) ) ;
#3705=SHAPE_DEFINITION_REPRESENTATION ( #3410, #573 ) ;
#3706=CARTESIAN_POINT ( 'NONE',  ( 12.49965553489658454, 48.41238076809164426, -11.67579978239260541 ) ) ;
#3716=CARTESIAN_POINT ( 'NONE',  ( -11.23255197390108506, 48.72302474870181044, -6.955105218463160099 ) ) ;
#3726=CARTESIAN_POINT ( 'NONE',  ( -9.126495132297684165, -49.16089547422079420, -21.05129937300930010 ) ) ;
#3736=CARTESIAN_POINT ( 'NONE',  ( 7.296436711415933196, -49.46595054402523317, -2.342244756090394286 ) ) ;
#3746=EDGE_CURVE ( 'NONE', #6887, #4209, #4934, .T. ) ;
#3767=CARTESIAN_POINT ( 'NONE',  ( -11.85818221415417284, 48.57454970542616479, -8.462724116359975568 ) ) ;
#3771=CARTESIAN_POINT ( 'NONE',  ( 0.000000000000000000, 0.000000000000000000, -250.0000000000000000 ) ) ;
#3776=CARTESIAN_POINT ( 'NONE',  ( -6.616553374552188949, -49.56145291835652245, -23.11303593919431165 ) ) ;
#3778=EDGE_LOOP ( 'NONE', ( #7280, #446 ) ) ;
#3784=CARTESIAN_POINT ( 'NONE',  ( 9.130470200569520856, -49.16013940401185067, -3.953130373342526926 ) ) ;
#3798=CARTESIAN_POINT ( 'NONE',  ( 6.266608689623135220, 49.60708521373746294, -23.32352924753791967 ) ) ;
#3801=DIRECTION ( 'NONE',  ( -0.000000000000000000, -7.945337353457666666E-18, -1.000000000000000000 ) ) ;
#3828=ORIENTED_EDGE ( 'NONE', *, *, #2977, .T. ) ;
#3842=CARTESIAN_POINT ( 'NONE',  ( -3.257004588345655982, 49.90043368416229441, -24.59660869042693676 ) ) ;
#3858=DIRECTION ( 'NONE',  ( 0.000000000000000000, 1.000000000000000000, 0.000000000000000000 ) ) ;
#3860=CARTESIAN_POINT ( 'NONE',  ( 0.000000000000000000, -49.99999999999999289, 0.000000000000000000 ) ) ;
#3875=EDGE_LOOP ( 'NONE', ( #8335, #996, #4449, #7820 ) ) ;
#3886=DIRECTION ( 'NONE',  ( 0.000000000000000000, 0.000000000000000000, 1.000000000000000000 ) ) ;
#3915=VERTEX_POINT ( 'NONE', #7904 ) ;
#3943=CIRCLE ( 'NONE', #6091, 2.499999999999996003 ) ;
#3963=CIRCLE ( 'NONE', #7346, 49.99999999999998579 ) ;
#4015=CIRCLE ( 'NONE', #4274, 3.000000000000001776 ) ;
#4021=VERTEX_POINT ( 'NONE', #6860 ) ;
#4039=CARTESIAN_POINT ( 'NONE',  ( 0.000000000000000000, 2.499999999999984013, -246.6833752096445664 ) ) ;
#4089=CYLINDRICAL_SURFACE ( 'NONE', #6569, 12.50000000000000000 ) ;
#4147=PRODUCT_DEFINITION ( 'UNKNOWN', '', #3524, #2933 ) ;
#4148=AXIS2_PLACEMENT_3D ( 'NONE', #6948, #1130, #3858 ) ;
#4176=CARTESIAN_POINT ( 'NONE',  ( -7.288983341925909798, -49.46703930816845940, -2.336970728266630548 ) ) ;
#4191=ORIENTED_EDGE ( 'NONE', *, *, #7217, .F. ) ;
#4197=CIRCLE ( 'NONE', #987, 12.50000000000000000 ) ;
#4208=AXIS2_PLACEMENT_3D ( 'NONE', #5026, #1885, #1838 ) ;
#4209=VERTEX_POINT ( 'NONE', #5881 ) ;
#4224=LINE ( 'NONE', #7465, #7210 ) ;
#4231=B_SPLINE_CURVE_WITH_KNOTS ( 'NONE', 3,
 ( #3001, #1627, #5592, #2350, #993, #4252, #8117, #4944, #1077, #4176, #3679, #341, #2391, #3582, #6256, #3539, #6119, #8168, #3631, #6169, #479, #2310, #7455, #5419, #7996, #7494, #2236, #1707, #7365, #4775, #1582, #3095, #3131, #1890, #5756, #4432, #3726, #1975, #3046, #3776, #7717, #5162, #6381, #4387, #522, #5678, #4993, #2598, #1798, #6346 ),
 .UNSPECIFIED., .F., .F.,
 ( 4, 2, 2, 2, 2, 2, 2, 2, 2, 2, 2, 2, 2, 2, 2, 2, 2, 2, 2, 2, 2, 2, 2, 2, 4 ),
 ( 0.000000000000000000, 0.002452303327911183745, 0.003678454991866776051, 0.004904606655822365754, 0.007356909983733550366, 0.008583061647689143106, 0.009809213311644733244, 0.01226151663955592046, 0.01348766830351151406, 0.01471381996746710594, 0.01593997163142269607, 0.01716612329537828968, 0.01961842662328948036, 0.02207072995120067452, 0.02452303327911185826, 0.02574918494306745534, 0.02697533660702304548, 0.02820148827097863561, 0.02942763993493422922, 0.03187994326284540603, 0.03310609492680098576, 0.03433224659075657242, 0.03678454991866773882, 0.03801070158262331855, 0.03923685324657889828 ),
 .UNSPECIFIED. ) ;
#4235=CARTESIAN_POINT ( 'NONE',  ( 7.288983341925910686, 49.46703930816845940, -2.336970728266630992 ) ) ;
#4252=CARTESIAN_POINT ( 'NONE',  ( -4.030269011847451566, -49.83886670901035387, -0.6603997896886458774 ) ) ;
#4263=CARTESIAN_POINT ( 'NONE',  ( 4.038684223623524083, -49.84236097863851711, -24.35762614583959618 ) ) ;
#4274=AXIS2_PLACEMENT_3D ( 'NONE', #3383, #2690, #5973 ) ;
#4277=LINE ( 'NONE', #5011, #2698 ) ;
#4295=CARTESIAN_POINT ( 'NONE',  ( 0.000000000000000000, -125.0000000000000000, -25.00000000000000000 ) ) ;
#4310=ADVANCED_FACE ( 'NONE', ( #5373 ), #4089, .T. ) ;
#4324=PRODUCT_CONTEXT ( 'NONE', #7154, 'mechanical' ) ;
#4347=DIRECTION ( 'NONE',  ( 0.000000000000000000, 1.000000000000000000, 0.000000000000000000 ) ) ;
#4352=CARTESIAN_POINT ( 'NONE',  ( 12.17681684015966503, -48.49465898589868118, -15.35333092327343785 ) ) ;
#4353=ADVANCED_FACE ( 'NONE', ( #1502 ), #7915, .T. ) ;
#4354=FACE_OUTER_BOUND ( 'NONE', #2071, .T. ) ;
#4373=ORIENTED_EDGE ( 'NONE', *, *, #5064, .F. ) ;
#4378=CARTESIAN_POINT ( 'NONE',  ( -5.536947881659091131, 49.69381142126947992, -23.71430020744633183 ) ) ;
#4382=DIRECTION ( 'NONE',  ( 0.000000000000000000, 1.000000000000000000, 0.000000000000000000 ) ) ;
#4387=CARTESIAN_POINT ( 'NONE',  ( -4.037232620646160619, -49.84250566375262537, -24.35825330067164174 ) ) ;
#4391=CARTESIAN_POINT ( 'NONE',  ( 0.8292248493948921606, -50.00000000000000711, -9.486769009248113261E-17 ) ) ;
#4392=DIRECTION ( 'NONE',  ( 0.000000000000000000, 1.000000000000000000, 0.000000000000000000 ) ) ;
#4393=VECTOR ( 'NONE', #263, 1000.000000000000000 ) ;
#4397=CARTESIAN_POINT ( 'NONE',  ( 4.592425496802573578E-15, -37.49999999999999289, -150.0000000000000000 ) ) ;
#4423=CARTESIAN_POINT ( 'NONE',  ( -5.167842669270958034, 49.73365441721957581, -23.88900650468791298 ) ) ;
#4425=FACE_OUTER_BOUND ( 'NONE', #5866, .T. ) ;
#4432=CARTESIAN_POINT ( 'NONE',  ( -9.403255565416666073, -49.10853579810842717, -20.74590799004609210 ) ) ;
#4440=CARTESIAN_POINT ( 'NONE',  ( 1.646459091894410642, -49.97939023862976882, -0.08171336424531111531 ) ) ;
#4447=ORIENTED_EDGE ( 'NONE', *, *, #680, .F. ) ;
#4449=ORIENTED_EDGE ( 'NONE', *, *, #2130, .T. ) ;
#4466=CARTESIAN_POINT ( 'NONE',  ( -7.631816331990290081, 49.41886753685898270, -22.43335506184081751 ) ) ;
#4481=CARTESIAN_POINT ( 'NONE',  ( 10.84023063519268071, -48.81293515762428115, -18.77686690299335481 ) ) ;
#4486=VERTEX_POINT ( 'NONE', #4295 ) ;
#4495=CARTESIAN_POINT ( 'NONE',  ( 9.403255565416678508, 49.10853579810846270, -20.74590799004608854 ) ) ;
#4502=CARTESIAN_POINT ( 'NONE',  ( -0.8175244905105707449, 50.00000000000000711, -25.00000000000000355 ) ) ;
#4520=LINE ( 'NONE', #1336, #2564 ) ;
#4525=ORIENTED_EDGE ( 'NONE', *, *, #4698, .T. ) ;
#4546=CARTESIAN_POINT ( 'NONE',  ( -7.627277604624987717, 49.41585025822053012, -2.588352797709350561 ) ) ;
#4549=PLANE ( 'NONE',  #1254 ) ;
#4552=DIRECTION ( 'NONE',  ( 0.000000000000000000, 1.000000000000000000, 0.000000000000000000 ) ) ;
#4582=EDGE_CURVE ( 'NONE', #1706, #6062, #1190, .T. ) ;
#4600=CARTESIAN_POINT ( 'NONE',  ( 0.000000000000000000, 1.986334338364416506E-15, 0.000000000000000000 ) ) ;
#4602=DIRECTION ( 'NONE',  ( -0.000000000000000000, -1.000000000000000000, -0.000000000000000000 ) ) ;
#4618=CARTESIAN_POINT ( 'NONE',  ( 0.000000000000000000, 0.000000000000000000, -248.3416876048222832 ) ) ;
#4619=ADVANCED_FACE ( 'NONE', ( #1203 ), #7142, .T. ) ;
#4620=EDGE_LOOP ( 'NONE', ( #392, #7089 ) ) ;
#4641=CARTESIAN_POINT ( 'NONE',  ( -1.646459091894399984, 49.97939023862978303, -0.08171336424531015774 ) ) ;
#4658=DIRECTION ( 'NONE',  ( -0.000000000000000000, -7.945337353457666666E-18, -1.000000000000000000 ) ) ;
#4667=CARTESIAN_POINT ( 'NONE',  ( 3.061616997868377718E-16, -2.499999999999995115, -150.0000000000000000 ) ) ;
#4675=EDGE_CURVE ( 'NONE', #6928, #6306, #1971, .T. ) ;
#4684=CARTESIAN_POINT ( 'NONE',  ( 0.000000000000000000, 1.191800603018649864E-15, -100.0000000000000000 ) ) ;
#4698=EDGE_CURVE ( 'NONE', #2803, #334, #5087, .T. ) ;
#4720=EDGE_CURVE ( 'NONE', #3915, #6329, #7834, .T. ) ;
#4725=DIRECTION ( 'NONE',  ( 0.000000000000000000, 1.000000000000000000, 0.000000000000000000 ) ) ;
#4734=ADVANCED_FACE ( 'NONE', ( #5988 ), #6711, .T. ) ;
#4737=CARTESIAN_POINT ( 'NONE',  ( 0.000000000000000000, 0.000000000000000000, -250.0000000000000000 ) ) ;
#4760=CARTESIAN_POINT ( 'NONE',  ( 6.271675211807171912, 49.60982880777384452, -1.656483108071705068 ) ) ;
#4775=CARTESIAN_POINT ( 'NONE',  ( -11.38780311525837163, -48.68618002971793146, -17.67075055658902016 ) ) ;
#4805=CARTESIAN_POINT ( 'NONE',  ( 6.123246359811209136E-15, -49.99999999999999289, -25.00000000000000000 ) ) ;
#4819=( NAMED_UNIT ( * ) PLANE_ANGLE_UNIT ( ) SI_UNIT ( $, .RADIAN. ) );
#4832=DIRECTION ( 'NONE',  ( 0.000000000000000000, 1.000000000000000000, 0.000000000000000000 ) ) ;
#4833=ADVANCED_FACE ( 'NONE', ( #5325 ), #3441, .T. ) ;
#4874=CIRCLE ( 'NONE', #5958, 12.50000000000000000 ) ;
#4923=CARTESIAN_POINT ( 'NONE',  ( 4.030269011847453342, 49.83886670901035387, -0.6603997896886467656 ) ) ;
#4933=PLANE ( 'NONE',  #5639 ) ;
#4934=CIRCLE ( 'NONE', #8180, 2.499999999999996003 ) ;
#4944=CARTESIAN_POINT ( 'NONE',  ( -5.554896158147707652, -49.69628058154707873, -1.272184882194882904 ) ) ;
#4971=CARTESIAN_POINT ( 'NONE',  ( 8.257771144136533792, 49.31688802671483529, -21.91964719072836587 ) ) ;
#4978=ORIENTED_EDGE ( 'NONE', *, *, #1413, .F. ) ;
#4987=CYLINDRICAL_SURFACE ( 'NONE', #4208, 12.50000000000000000 ) ;
#4993=CARTESIAN_POINT ( 'NONE',  ( -1.638770961094136114, -49.97482151629360914, -24.89896468147090758 ) ) ;
#5011=CARTESIAN_POINT ( 'NONE',  ( 0.000000000000000000, 2.499999999999990230, -250.0000000000000000 ) ) ;
#5017=CARTESIAN_POINT ( 'NONE',  ( 1.530808498934191521E-15, -125.0000000000000000, 0.000000000000000000 ) ) ;
#5026=CARTESIAN_POINT ( 'NONE',  ( 0.000000000000000000, 125.0000000000000000, -12.50000000000000000 ) ) ;
#5029=PLANE ( 'NONE',  #7006 ) ;
#5043=CARTESIAN_POINT ( 'NONE',  ( 3.256071768936471766, -49.89543388580304395, -0.4244881437574537508 ) ) ;
#5044=DIRECTION ( 'NONE',  ( -0.000000000000000000, -7.945337353457666666E-18, -1.000000000000000000 ) ) ;
#5047=ORIENTED_EDGE ( 'NONE', *, *, #4675, .F. ) ;
#5049=ORIENTED_EDGE ( 'NONE', *, *, #737, .T. ) ;
#5055=CARTESIAN_POINT ( 'NONE',  ( 9.920587673301477949, 49.00664693364542046, -20.11565191071547787 ) ) ;
#5064=EDGE_CURVE ( 'NONE', #334, #2803, #1881, .T. ) ;
#5066=CARTESIAN_POINT ( 'NONE',  ( -9.130470200569520856, 49.16013940401185778, -3.953130373342527815 ) ) ;
#5075=FACE_BOUND ( 'NONE', #4620, .T. ) ;
#5080=DIRECTION ( 'NONE',  ( 0.000000000000000000, 1.000000000000000000, 0.000000000000000000 ) ) ;
#5081=CARTESIAN_POINT ( 'NONE',  ( 11.23255197390109217, -48.72302474870180333, -6.955105218463169869 ) ) ;
#5087=CIRCLE ( 'NONE', #8204, 2.499999999999984013 ) ;
#5098=CARTESIAN_POINT ( 'NONE',  ( 10.61457161467473398, 48.86086578770957800, -19.11406644883056316 ) ) ;
#5110=CARTESIAN_POINT ( 'NONE',  ( -1.632468168883555837, 49.97996006834706151, -24.92059050027006606 ) ) ;
#5119=CARTESIAN_POINT ( 'NONE',  ( 0.000000000000000000, 37.50000000000000000, -100.0000000000000000 ) ) ;
#5126=CARTESIAN_POINT ( 'NONE',  ( 12.47905948369885998, -48.41771210405730130, -13.33173448961934504 ) ) ;
#5142=CARTESIAN_POINT ( 'NONE',  ( 1.638770961094149436, 49.97482151629360203, -24.89896468147090403 ) ) ;
#5147=VERTEX_POINT ( 'NONE', #5017 ) ;
#5154=CARTESIAN_POINT ( 'NONE',  ( -12.07731880710695904, 48.51961889015782958, -15.74894529186713221 ) ) ;
#5162=CARTESIAN_POINT ( 'NONE',  ( -5.541544814107227879, -49.69330507166043276, -23.71206720076232699 ) ) ;
#5165=ORIENTED_EDGE ( 'NONE', *, *, #5679, .F. ) ;
#5197=CARTESIAN_POINT ( 'NONE',  ( 4.592425496802574367E-15, -37.50000000000000000, -100.0000000000000000 ) ) ;
#5212=CARTESIAN_POINT ( 'NONE',  ( 9.920332936303610794, -49.00669811220510041, -4.884022838024439928 ) ) ;
#5219=APPLICATION_CONTEXT ( 'automotive_design' ) ;
#5227=CYLINDRICAL_SURFACE ( 'NONE', #2027, 12.50000000000000000 ) ;
#5239=DIRECTION ( 'NONE',  ( 0.000000000000000000, 1.000000000000000000, 0.000000000000000000 ) ) ;
#5285=CARTESIAN_POINT ( 'NONE',  ( 0.000000000000000000, 0.000000000000000000, -250.0000000000000000 ) ) ;
#5308=ORIENTED_EDGE ( 'NONE', *, *, #3547, .T. ) ;
#5324=PRODUCT ( 'Probe', 'Probe', '', ( #4324 ) ) ;
#5325=FACE_OUTER_BOUND ( 'NONE', #1747, .T. ) ;
#5373=FACE_OUTER_BOUND ( 'NONE', #2761, .T. ) ;
#5419=CARTESIAN_POINT ( 'NONE',  ( -12.41960978562213924, -48.43326235599739249, -10.86247626165360636 ) ) ;
#5448=PLANE ( 'NONE',  #457 ) ;
#5453=B_SPLINE_CURVE_WITH_KNOTS ( 'NONE', 3,
 ( #281, #2944, #3611, #5534, #7978, #4923, #2896, #6707, #4760, #4235, #7393, #242, #2820, #936, #6754, #3520, #1058, #6103, #327, #5574, #3142, #2462, #5698, #2501, #3706, #1957, #551, #8190, #3118, #7650, #3194, #7005, #5098, #2581, #5055, #4495, #1781, #4971, #1865, #8322, #3798, #7606, #2418, #592, #3073, #7696, #5142, #7563, #1912, #8283 ),
 .UNSPECIFIED., .F., .F.,
 ( 4, 2, 2, 2, 2, 2, 2, 2, 2, 2, 2, 2, 2, 2, 2, 2, 2, 2, 2, 2, 2, 2, 2, 2, 4 ),
 ( 1.991839973943360954E-18, 0.002452303327911185479, 0.003678454991866776918, 0.004904606655822368357, 0.007356909983733552968, 0.008583061647689146575, 0.009809213311644738448, 0.01226151663955592219, 0.01348766830351151233, 0.01471381996746710420, 0.01593997163142269261, 0.01716612329537827927, 0.01961842662328945261, 0.02207072995120062595, 0.02452303327911179581, 0.02574918494306738595, 0.02697533660702297262, 0.02820148827097856276, 0.02942763993493414942, 0.03187994326284532970, 0.03310609492680091637, 0.03433224659075650997, 0.03678454991866769025, 0.03801070158262329080, 0.03923685324657887746 ),
 .UNSPECIFIED. ) ;
#5524=CIRCLE ( 'NONE', #6604, 3.000000000000002665 ) ;
#5525=EDGE_LOOP ( 'NONE', ( #3147, #1069, #4191, #182, #856, #6799 ) ) ;
#5534=CARTESIAN_POINT ( 'NONE',  ( 2.846087801003402529, 49.92054308009031161, -0.3214687869884013671 ) ) ;
#5572=EDGE_LOOP ( 'NONE', ( #4447, #3828, #3381, #2786 ) ) ;
#5574=CARTESIAN_POINT ( 'NONE',  ( 11.69960264931230043, 48.61219013327713157, -8.080179916824185682 ) ) ;
#5592=CARTESIAN_POINT ( 'NONE',  ( -1.644392415218294268, -49.97938897499117417, -0.08173415109641084253 ) ) ;
#5599=CARTESIAN_POINT ( 'NONE',  ( 6.123233995736765296E-15, -49.99999999999998579, -100.0000000000000000 ) ) ;
#5601=DIRECTION ( 'NONE',  ( -1.000000000000000000, -0.000000000000000000, 0.000000000000000000 ) ) ;
#5639=AXIS2_PLACEMENT_3D ( 'NONE', #7084, #7737, #6934 ) ;
#5663=CARTESIAN_POINT ( 'NONE',  ( 0.000000000000000000, 50.00000000000000000, 0.000000000000000000 ) ) ;
#5669=CARTESIAN_POINT ( 'NONE',  ( -9.920332936303609017, 49.00669811220510752, -4.884022838024439039 ) ) ;
#5678=CARTESIAN_POINT ( 'NONE',  ( -2.050159205374797455, -49.95957628852639942, -24.83755891087360013 ) ) ;
#5679=EDGE_CURVE ( 'NONE', #986, #6306, #6448, .T. ) ;
#5683=CARTESIAN_POINT ( 'NONE',  ( 9.400408038818898859, -49.10908733398244408, -20.74923976180173213 ) ) ;
#5698=CARTESIAN_POINT ( 'NONE',  ( 12.17797428566710138, 48.49436920628651393, -9.651054563031580713 ) ) ;
#5705=CARTESIAN_POINT ( 'NONE',  ( -12.47905948369886353, 48.41771210405730130, -13.33173448961933794 ) ) ;
#5713=EDGE_CURVE ( 'NONE', #334, #4021, #4015, .T. ) ;
#5724=CARTESIAN_POINT ( 'NONE',  ( 0.000000000000000000, 7.945337353457666419E-16, -150.0000000000000000 ) ) ;
#5756=CARTESIAN_POINT ( 'NONE',  ( -9.920587673301467291, -49.00664693364539914, -20.11565191071548142 ) ) ;
#5767=CARTESIAN_POINT ( 'NONE',  ( 7.631816331990286528, -49.41886753685898270, -22.43335506184081751 ) ) ;
#5809=CARTESIAN_POINT ( 'NONE',  ( 8.256742446866514484, -49.31458024324042810, -3.106261761854192560 ) ) ;
#5811=DIRECTION ( 'NONE',  ( 0.000000000000000000, -1.000000000000000000, 0.000000000000000000 ) ) ;
#5824=EDGE_LOOP ( 'NONE', ( #6809, #7520 ) ) ;
#5847=AXIS2_PLACEMENT_3D ( 'NONE', #4737, #7409, #1540 ) ;
#5848=CARTESIAN_POINT ( 'NONE',  ( 11.85818221415417462, -48.57454970542615769, -8.462724116359982673 ) ) ;
#5866=EDGE_LOOP ( 'NONE', ( #7425, #5049, #418, #3312 ) ) ;
#5868=CARTESIAN_POINT ( 'NONE',  ( -3.256071768936462885, 49.89543388580307948, -0.4244881437574492544 ) ) ;
#5874=CIRCLE ( 'NONE', #7225, 37.49999999999999289 ) ;
#5881=CARTESIAN_POINT ( 'NONE',  ( 0.000000000000000000, 2.499999999999996891, -150.0000000000000000 ) ) ;
#5884=CARTESIAN_POINT ( 'NONE',  ( 0.000000000000000000, 0.000000000000000000, 0.000000000000000000 ) ) ;
#5890=AXIS2_PLACEMENT_3D ( 'NONE', #39, #3165, #4552 ) ;
#5895=DIRECTION ( 'NONE',  ( -0.000000000000000000, -1.000000000000000000, -0.000000000000000000 ) ) ;
#5905=CARTESIAN_POINT ( 'NONE',  ( -2.854599402353548587, 49.92007443197289263, -0.3233859435660823567 ) ) ;
#5927=DIRECTION ( 'NONE',  ( 1.000000000000000000, 0.000000000000000000, 0.000000000000000000 ) ) ;
#5958=AXIS2_PLACEMENT_3D ( 'NONE', #1947, #1384, #6524 ) ;
#5962=CARTESIAN_POINT ( 'NONE',  ( 0.000000000000000000, 125.0000000000000000, -12.50000000000000000 ) ) ;
#5973=DIRECTION ( 'NONE',  ( 1.224646799147353207E-16, -1.000000000000000000, 0.000000000000000000 ) ) ;
#5988=FACE_OUTER_BOUND ( 'NONE', #5525, .T. ) ;
#6006=MECHANICAL_DESIGN_GEOMETRIC_PRESENTATION_REPRESENTATION('',(#2901),#6967);
#6026=DIRECTION ( 'NONE',  ( -0.000000000000000000, -1.000000000000000000, -0.000000000000000000 ) ) ;
#6052=ORIENTED_EDGE ( 'NONE', *, *, #6250, .T. ) ;
#6062=VERTEX_POINT ( 'NONE', #484 ) ;
#6064=CARTESIAN_POINT ( 'NONE',  ( 0.000000000000000000, 0.000000000000000000, -248.3416876048222832 ) ) ;
#6084=ORIENTED_EDGE ( 'NONE', *, *, #8043, .F. ) ;
#6091=AXIS2_PLACEMENT_3D ( 'NONE', #526, #997, #1035 ) ;
#6103=CARTESIAN_POINT ( 'NONE',  ( 11.21327906667868390, 48.72680251680211683, -6.961169940684509783 ) ) ;
#6118=ORIENTED_EDGE ( 'NONE', *, *, #7448, .F. ) ;
#6119=CARTESIAN_POINT ( 'NONE',  ( -10.82846484896509232, -48.81376096915063556, -6.242155733168281095 ) ) ;
#6153=ORIENTED_EDGE ( 'NONE', *, *, #135, .T. ) ;
#6169=CARTESIAN_POINT ( 'NONE',  ( -11.69960264931230220, -48.61219013327713157, -8.080179916824185682 ) ) ;
#6172=ORIENTED_EDGE ( 'NONE', *, *, #3547, .F. ) ;
#6204=EDGE_LOOP ( 'NONE', ( #775, #2507, #2710 ) ) ;
#6205=DIRECTION ( 'NONE',  ( 0.000000000000000000, 0.000000000000000000, 1.000000000000000000 ) ) ;
#6216=ORIENTED_EDGE ( 'NONE', *, *, #4720, .T. ) ;
#6225=AXIS2_PLACEMENT_3D ( 'NONE', #5285, #7866, #6587 ) ;
#6250=EDGE_CURVE ( 'NONE', #4486, #5147, #2692, .T. ) ;
#6256=CARTESIAN_POINT ( 'NONE',  ( -9.931622870156765259, -49.00592830463494209, -4.865363096503712903 ) ) ;
#6264=CARTESIAN_POINT ( 'NONE',  ( 5.167842669270961586, -49.73365441721959002, -23.88900650468791298 ) ) ;
#6290=CARTESIAN_POINT ( 'NONE',  ( -10.84905357516155711, 48.81101040073316710, -6.237423197851057921 ) ) ;
#6306=VERTEX_POINT ( 'NONE', #5663 ) ;
#6313=CARTESIAN_POINT ( 'NONE',  ( 4.044723210857163131, -49.83770199522206212, -0.6652966195906406810 ) ) ;
#6318=DIRECTION ( 'NONE',  ( 0.000000000000000000, -1.000000000000000000, 0.000000000000000000 ) ) ;
#6329=VERTEX_POINT ( 'NONE', #8198 ) ;
#6336=ORIENTED_EDGE ( 'NONE', *, *, #721, .F. ) ;
#6344=DIRECTION ( 'NONE',  ( 0.000000000000000000, -1.000000000000000000, 7.945337353457666666E-18 ) ) ;
#6346=CARTESIAN_POINT ( 'NONE',  ( 6.123246359811209136E-15, -49.99999999999999289, -25.00000000000000000 ) ) ;
#6352=CARTESIAN_POINT ( 'NONE',  ( 0.000000000000000000, 1.191800603018649864E-15, -100.0000000000000000 ) ) ;
#6353=CARTESIAN_POINT ( 'NONE',  ( 11.83910760917652105, -48.57829327830486221, -16.53147691254503826 ) ) ;
#6376=CARTESIAN_POINT ( 'NONE',  ( 0.000000000000000000, 2.635170283421476540E-17, -246.6833752096445664 ) ) ;
#6381=CARTESIAN_POINT ( 'NONE',  ( -5.169052467613977520, -49.73353547763984039, -23.88849205255370123 ) ) ;
#6387=FACE_OUTER_BOUND ( 'NONE', #5572, .T. ) ;
#6407=CARTESIAN_POINT ( 'NONE',  ( -10.16267929626374666, 48.95685099404312979, -19.78936650929338370 ) ) ;
#6426=CARTESIAN_POINT ( 'NONE',  ( 12.33692650994068174, -48.45417487488280983, -14.55343858072928676 ) ) ;
#6448=CIRCLE ( 'NONE', #2037, 50.00000000000000000 ) ;
#6457=CARTESIAN_POINT ( 'NONE',  ( -12.39753912377990019, 48.43864980223352745, -14.14916085730399331 ) ) ;
#6472=DIRECTION ( 'NONE',  ( -0.000000000000000000, -7.945337353457666666E-18, -1.000000000000000000 ) ) ;
#6521=ADVANCED_BREP_SHAPE_REPRESENTATION ( '', ( #3583, #1299 ), #7094 ) ;
#6524=DIRECTION ( 'NONE',  ( 0.000000000000000000, 0.000000000000000000, 1.000000000000000000 ) ) ;
#6560=EDGE_CURVE ( 'NONE', #2803, #4021, #5524, .T. ) ;
#6569=AXIS2_PLACEMENT_3D ( 'NONE', #5962, #2185, #861 ) ;
#6587=DIRECTION ( 'NONE',  ( 0.000000000000000000, 1.000000000000000000, 0.000000000000000000 ) ) ;
#6589=ORIENTED_EDGE ( 'NONE', *, *, #5713, .T. ) ;
#6604=AXIS2_PLACEMENT_3D ( 'NONE', #6064, #2256, #3020 ) ;
#6652=CARTESIAN_POINT ( 'NONE',  ( 0.000000000000000000, -2.761866872635923494E-33, -100.0000000000000000 ) ) ;
#6653=CLOSED_SHELL ( 'NONE', ( #6966, #188, #4619, #2578, #19, #4734, #4353, #1237, #2715, #1157, #1437, #7162, #7752, #3025, #4310, #4833, #496 ) ) ;
#6668=CARTESIAN_POINT ( 'NONE',  ( 0.000000000000000000, 7.945337353457666419E-16, -150.0000000000000000 ) ) ;
#6675=FACE_OUTER_BOUND ( 'NONE', #3778, .T. ) ;
#6700=ORIENTED_EDGE ( 'NONE', *, *, #1915, .T. ) ;
#6707=CARTESIAN_POINT ( 'NONE',  ( 5.554896158147704988, 49.69628058154707162, -1.272184882194884903 ) ) ;
#6711=CYLINDRICAL_SURFACE ( 'NONE', #7121, 49.99999999999999289 ) ;
#6733=FACE_BOUND ( 'NONE', #1746, .T. ) ;
#6754=CARTESIAN_POINT ( 'NONE',  ( 9.931622870156768812, 49.00592830463494920, -4.865363096503712903 ) ) ;
#6795=DIRECTION ( 'NONE',  ( 0.000000000000000000, 1.000000000000000000, 0.000000000000000000 ) ) ;
#6799=ORIENTED_EDGE ( 'NONE', *, *, #1655, .T. ) ;
#6809=ORIENTED_EDGE ( 'NONE', *, *, #8282, .T. ) ;
#6817=LINE ( 'NONE', #8126, #2043 ) ;
#6847=VECTOR ( 'NONE', #7665, 1000.000000000000000 ) ;
#6856=EDGE_LOOP ( 'NONE', ( #5165, #8249 ) ) ;
#6860=CARTESIAN_POINT ( 'NONE',  ( 0.000000000000000000, -2.075330319324761228E-16, -251.3416876048222832 ) ) ;
#6887=VERTEX_POINT ( 'NONE', #4667 ) ;
#6927=ORIENTED_EDGE ( 'NONE', *, *, #721, .T. ) ;
#6928=VERTEX_POINT ( 'NONE', #7168 ) ;
#6934=DIRECTION ( 'NONE',  ( 0.000000000000000000, -0.000000000000000000, 1.000000000000000000 ) ) ;
#6948=CARTESIAN_POINT ( 'NONE',  ( 0.000000000000000000, 0.000000000000000000, -250.0000000000000000 ) ) ;
#6966=ADVANCED_FACE ( 'NONE', ( #2694 ), #5227, .T. ) ;
#6967=( GEOMETRIC_REPRESENTATION_CONTEXT ( 3 ) GLOBAL_UNCERTAINTY_ASSIGNED_CONTEXT ( ( #491 ) ) GLOBAL_UNIT_ASSIGNED_CONTEXT ( ( #6982, #8296, #7062 ) ) REPRESENTATION_CONTEXT ( 'NONE', 'WORKASPACE' ) );
#6980=DIRECTION ( 'NONE',  ( 0.000000000000000000, 7.945337353457666666E-18, 1.000000000000000000 ) ) ;
#6982=( LENGTH_UNIT ( ) NAMED_UNIT ( * ) SI_UNIT ( .MILLI., .METRE. ) );
#7005=CARTESIAN_POINT ( 'NONE',  ( 10.82421258667008246, 48.81470695058815323, -18.76526308057256287 ) ) ;
#7006=AXIS2_PLACEMENT_3D ( 'NONE', #1888, #6980, #6344 ) ;
#7017=CARTESIAN_POINT ( 'NONE',  ( -12.50025679328619077, 48.41222552385477229, -11.67941733774922142 ) ) ;
#7033=CARTESIAN_POINT ( 'NONE',  ( 11.69966253144280799, -48.61218256317028619, -16.92010850872652128 ) ) ;
#7053=CARTESIAN_POINT ( 'NONE',  ( -9.400408038818907741, 49.10908733398244408, -20.74923976180172858 ) ) ;
#7059=DIRECTION ( 'NONE',  ( 0.000000000000000000, 1.000000000000000000, 0.000000000000000000 ) ) ;
#7062=( NAMED_UNIT ( * ) SI_UNIT ( $, .STERADIAN. ) SOLID_ANGLE_UNIT ( ) );
#7071=CARTESIAN_POINT ( 'NONE',  ( 12.49987068959938341, -48.41232521539284051, -12.91614503987825735 ) ) ;
#7081=EDGE_CURVE ( 'NONE', #3598, #6062, #6817, .T. ) ;
#7084=CARTESIAN_POINT ( 'NONE',  ( 0.000000000000000000, -125.0000000000000000, -12.50000000000000000 ) ) ;
#7089=ORIENTED_EDGE ( 'NONE', *, *, #3746, .F. ) ;
#7094=( GEOMETRIC_REPRESENTATION_CONTEXT ( 3 ) GLOBAL_UNCERTAINTY_ASSIGNED_CONTEXT ( ( #3110 ) ) GLOBAL_UNIT_ASSIGNED_CONTEXT ( ( #2351, #4819, #2960 ) ) REPRESENTATION_CONTEXT ( 'NONE', 'WORKASPACE' ) );
#7095=CARTESIAN_POINT ( 'NONE',  ( -4.038684223623520531, 49.84236097863853132, -24.35762614583960683 ) ) ;
#7116=CARTESIAN_POINT ( 'NONE',  ( 10.84905357516155888, -48.81101040073316710, -6.237423197851056145 ) ) ;
#7121=AXIS2_PLACEMENT_3D ( 'NONE', #7180, #941, #1527 ) ;
#7126=VERTEX_POINT ( 'NONE', #5599 ) ;
#7140=CARTESIAN_POINT ( 'NONE',  ( 0.000000000000000000, -2.590378953665082788E-32, -3.260250431704825048E-15 ) ) ;
#7142=CYLINDRICAL_SURFACE ( 'NONE', #2414, 37.49999999999999289 ) ;
#7154=APPLICATION_CONTEXT ( 'automotive_design' ) ;
#7162=ADVANCED_FACE ( 'NONE', ( #6387 ), #1895, .T. ) ;
#7168=CARTESIAN_POINT ( 'NONE',  ( 1.530808498934191521E-15, 125.0000000000000000, 0.000000000000000000 ) ) ;
#7180=CARTESIAN_POINT ( 'NONE',  ( 0.000000000000000000, 0.000000000000000000, -250.0000000000000000 ) ) ;
#7210=VECTOR ( 'NONE', #3510, 1000.000000000000000 ) ;
#7217=EDGE_CURVE ( 'NONE', #7967, #7126, #1072, .T. ) ;
#7225=AXIS2_PLACEMENT_3D ( 'NONE', #5724, #5044, #4392 ) ;
#7243=FACE_OUTER_BOUND ( 'NONE', #435, .T. ) ;
#7280=ORIENTED_EDGE ( 'NONE', *, *, #1024, .T. ) ;
#7303=ORIENTED_EDGE ( 'NONE', *, *, #7448, .T. ) ;
#7310=CARTESIAN_POINT ( 'NONE',  ( 0.000000000000000000, 49.99999999999998579, -100.0000000000000000 ) ) ;
#7346=AXIS2_PLACEMENT_3D ( 'NONE', #2250, #3469, #4832 ) ;
#7365=CARTESIAN_POINT ( 'NONE',  ( -11.86014387961075833, -48.57408496170467771, -16.53260109561407276 ) ) ;
#7393=CARTESIAN_POINT ( 'NONE',  ( 7.620025376658134952, 49.41698073774414013, -2.582688914155140125 ) ) ;
#7397=DIRECTION ( 'NONE',  ( -0.000000000000000000, -7.945337353457666666E-18, -1.000000000000000000 ) ) ;
#7409=DIRECTION ( 'NONE',  ( -0.000000000000000000, -7.945337353457666666E-18, -1.000000000000000000 ) ) ;
#7419=ORIENTED_EDGE ( 'NONE', *, *, #917, .T. ) ;
#7425=ORIENTED_EDGE ( 'NONE', *, *, #3367, .T. ) ;
#7448=EDGE_CURVE ( 'NONE', #6887, #2803, #4520, .T. ) ;
#7455=CARTESIAN_POINT ( 'NONE',  ( -12.17797428566710316, -48.49436920628652103, -9.651054563031587819 ) ) ;
#7465=CARTESIAN_POINT ( 'NONE',  ( 1.530808498934191521E-15, 125.0000000000000000, 0.000000000000000000 ) ) ;
#7485=DIRECTION ( 'NONE',  ( 0.000000000000000000, 1.000000000000000000, 0.000000000000000000 ) ) ;
#7494=CARTESIAN_POINT ( 'NONE',  ( -12.50034226774478441, -48.41220345444931183, -13.31371842734951727 ) ) ;
#7500=CARTESIAN_POINT ( 'NONE',  ( 3.257004588345654206, -49.90043368416228731, -24.59660869042692966 ) ) ;
#7501=CYLINDRICAL_SURFACE ( 'NONE', #5847, 2.499999999999990230 ) ;
#7520=ORIENTED_EDGE ( 'NONE', *, *, #4582, .T. ) ;
#7522=FACE_OUTER_BOUND ( 'NONE', #843, .T. ) ;
#7563=CARTESIAN_POINT ( 'NONE',  ( 0.8183949479883679823, 49.99498560413270098, -24.97998898815200164 ) ) ;
#7595=CIRCLE ( 'NONE', #2090, 50.00000000000000000 ) ;
#7606=CARTESIAN_POINT ( 'NONE',  ( 5.541544814107237649, 49.69330507166041144, -23.71206720076230923 ) ) ;
#7614=CARTESIAN_POINT ( 'NONE',  ( -12.33692650994067463, 48.45417487488279562, -14.55343858072927432 ) ) ;
#7617=EDGE_LOOP ( 'NONE', ( #739, #7303, #4373, #6084 ) ) ;
#7631=CARTESIAN_POINT ( 'NONE',  ( 6.274835263354066939, -49.60946935866542162, -1.658027691731849496 ) ) ;
#7634=EDGE_LOOP ( 'NONE', ( #6118, #8112, #2647, #1641 ) ) ;
#7650=CARTESIAN_POINT ( 'NONE',  ( 11.38780311525837696, 48.68618002971793146, -17.67075055658902372 ) ) ;
#7659=CARTESIAN_POINT ( 'NONE',  ( -8.557270319823464533, 49.26314968593495536, -3.379276828450693770 ) ) ;
#7665=DIRECTION ( 'NONE',  ( -0.000000000000000000, -1.000000000000000000, -0.000000000000000000 ) ) ;
#7696=CARTESIAN_POINT ( 'NONE',  ( 2.050159205374804561, 49.95957628852642074, -24.83755891087361078 ) ) ;
#7707=CARTESIAN_POINT ( 'NONE',  ( -6.614448519079573430, 49.56174273647123130, -23.11440585317445695 ) ) ;
#7717=CARTESIAN_POINT ( 'NONE',  ( -6.266608689623121897, -49.60708521373747715, -23.32352924753793033 ) ) ;
#7726=CARTESIAN_POINT ( 'NONE',  ( 7.627277604625000151, -49.41585025822053723, -2.588352797709359887 ) ) ;
#7737=DIRECTION ( 'NONE',  ( 0.000000000000000000, 1.000000000000000000, 0.000000000000000000 ) ) ;
#7752=ADVANCED_FACE ( 'NONE', ( #5075, #2999 ), #5029, .F. ) ;
#7764=CARTESIAN_POINT ( 'NONE',  ( 4.429756409623588631, -49.80481938051303814, -0.8041353051610896641 ) ) ;
#7771=ORIENTED_EDGE ( 'NONE', *, *, #1024, .F. ) ;
#7820=ORIENTED_EDGE ( 'NONE', *, *, #4720, .F. ) ;
#7834=LINE ( 'NONE', #3398, #7930 ) ;
#7855=ORIENTED_EDGE ( 'NONE', *, *, #6560, .F. ) ;
#7866=DIRECTION ( 'NONE',  ( -0.000000000000000000, -7.945337353457666666E-18, -1.000000000000000000 ) ) ;
#7879=SPHERICAL_SURFACE ( 'NONE', #222, 3.000000000000001776 ) ;
#7888=DIRECTION ( 'NONE',  ( 0.000000000000000000, -7.945337353457666666E-18, -1.000000000000000000 ) ) ;
#7904=CARTESIAN_POINT ( 'NONE',  ( 0.000000000000000000, 125.0000000000000000, -25.00000000000000000 ) ) ;
#7905=CARTESIAN_POINT ( 'NONE',  ( -4.429756409623576197, 49.80481938051305235, -0.8041353051610855562 ) ) ;
#7915=CYLINDRICAL_SURFACE ( 'NONE', #2916, 49.99999999999999289 ) ;
#7916=CARTESIAN_POINT ( 'NONE',  ( 4.592425496802573578E-15, -37.49999999999999289, -250.0000000000000000 ) ) ;
#7930=VECTOR ( 'NONE', #4602, 1000.000000000000000 ) ;
#7939=CARTESIAN_POINT ( 'NONE',  ( 0.000000000000000000, 50.00000000000000000, 0.000000000000000000 ) ) ;
#7949=DIRECTION ( 'NONE',  ( -0.000000000000000000, -7.945337353457666666E-18, -1.000000000000000000 ) ) ;
#7962=CARTESIAN_POINT ( 'NONE',  ( 3.061616997868367857E-16, -2.499999999999984013, -246.6833752096445664 ) ) ;
#7967=VERTEX_POINT ( 'NONE', #7310 ) ;
#7978=CARTESIAN_POINT ( 'NONE',  ( 3.243174531372581271, 49.89626761698125534, -0.4210505255250476808 ) ) ;
#7982=CARTESIAN_POINT ( 'NONE',  ( 0.000000000000000000, 125.0000000000000000, -12.50000000000000000 ) ) ;
#7987=AXIS2_PLACEMENT_3D ( 'NONE', #6652, #7888, #791 ) ;
#7996=CARTESIAN_POINT ( 'NONE',  ( -12.49965553489658276, -48.41238076809165136, -11.67579978239260541 ) ) ;
#8022=LINE ( 'NONE', #3443, #1412 ) ;
#8043=EDGE_CURVE ( 'NONE', #4209, #334, #4277, .T. ) ;
#8109=CARTESIAN_POINT ( 'NONE',  ( 0.000000000000000000, 125.0000000000000000, -12.50000000000000000 ) ) ;
#8112=ORIENTED_EDGE ( 'NONE', *, *, #3746, .T. ) ;
#8117=CARTESIAN_POINT ( 'NONE',  ( -4.420576121828486471, -49.80565028682020312, -0.8005904993895454069 ) ) ;
#8126=CARTESIAN_POINT ( 'NONE',  ( 0.000000000000000000, 37.49999999999999289, -250.0000000000000000 ) ) ;
#8129=FACE_OUTER_BOUND ( 'NONE', #7617, .T. ) ;
#8168=CARTESIAN_POINT ( 'NONE',  ( -11.21327906667868390, -48.72680251680210972, -6.961169940684510671 ) ) ;
#8180=AXIS2_PLACEMENT_3D ( 'NONE', #6668, #2213, #5239 ) ;
#8190=CARTESIAN_POINT ( 'NONE',  ( 12.09737906851130873, 48.51474822866214964, -15.75174765218249284 ) ) ;
#8198=CARTESIAN_POINT ( 'NONE',  ( -1.236408833568031405E-20, 49.99999999999999289, -25.00000000000000000 ) ) ;
#8201=CARTESIAN_POINT ( 'NONE',  ( -12.49987068959938519, 48.41232521539285472, -12.91614503987825024 ) ) ;
#8204=AXIS2_PLACEMENT_3D ( 'NONE', #6376, #2470, #4382 ) ;
#8248=CARTESIAN_POINT ( 'NONE',  ( -11.22541203495697815, 48.72469304432832615, -18.06039341770851436 ) ) ;
#8249=ORIENTED_EDGE ( 'NONE', *, *, #1655, .F. ) ;
#8266=CARTESIAN_POINT ( 'NONE',  ( 2.854599402353564130, -49.92007443197287841, -0.3233859435660855763 ) ) ;
#8282=EDGE_CURVE ( 'NONE', #6062, #1706, #5874, .T. ) ;
#8283=CARTESIAN_POINT ( 'NONE',  ( -1.236408833568031405E-20, 49.99999999999999289, -25.00000000000000000 ) ) ;
#8296=( NAMED_UNIT ( * ) PLANE_ANGLE_UNIT ( ) SI_UNIT ( $, .RADIAN. ) );
#8311=CIRCLE ( 'NONE', #1028, 12.50000000000000000 ) ;
#8322=CARTESIAN_POINT ( 'NONE',  ( 6.616553374552193389, 49.56145291835650823, -23.11303593919430099 ) ) ;
#8335=ORIENTED_EDGE ( 'NONE', *, *, #1545, .F. ) ;
#8387=COLOUR_RGB('Sky Blue',0.24,0.69,0.87);
#8388=FILL_AREA_STYLE_COLOUR('',#8387);
#8389=FILL_AREA_STYLE('',(#8388));
#8390=SURFACE_STYLE_FILL_AREA(#8389);
#8391=SURFACE_SIDE_STYLE('',(#8390));
#8392=SURFACE_STYLE_USAGE(.BOTH.,#8391);
#8393=PRESENTATION_STYLE_ASSIGNMENT((#8392));
ENDSEC;
END-ISO-10303-21;
